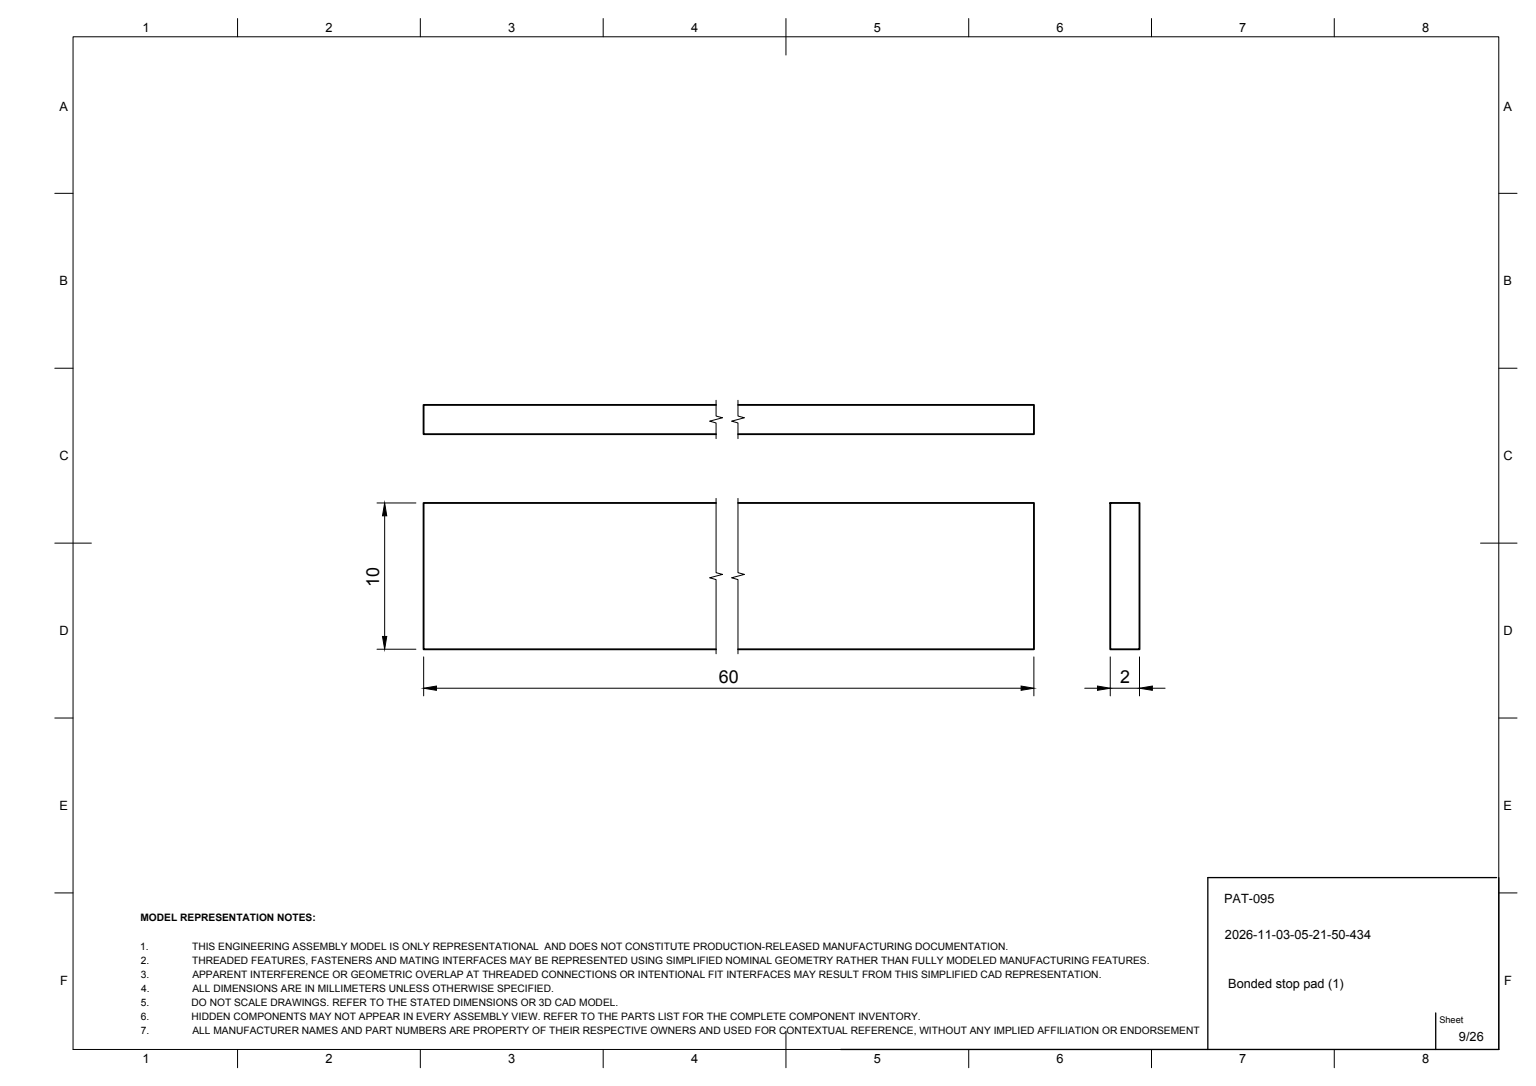
ISO-10303-21;
HEADER;
/* Generated by software containing ST-Developer
 * from STEP Tools, Inc. (www.steptools.com) 
 */

FILE_DESCRIPTION(
/* description */ ('Single-Axis Profile-Rail Linear Slide'),
/* implementation_level */ '2;1');

FILE_NAME(
/* name */ 'Bonded stop pad (1).step',
/* time_stamp */ '2026-10-27T10:47:43-07:00',
/* author */ (''),
/* organization */ (''),
/* preprocessor_version */ 'ST-DEVELOPER v20.2',
/* originating_system */ 'Autodesk Translation Framework v15.17.0.0',
/* authorisation */ '');

FILE_SCHEMA (('AUTOMOTIVE_DESIGN { 1 0 10303 214 3 1 1 }'));
ENDSEC;

DATA;
#10=MECHANICAL_DESIGN_GEOMETRIC_PRESENTATION_REPRESENTATION('',(#333),#14478);
#279=SHAPE_REPRESENTATION_RELATIONSHIP('SRR','None',#14609,#306);
#306=ADVANCED_BREP_SHAPE_REPRESENTATION('',(#360),#14453);
#333=STYLED_ITEM('',(#14845),#360);
#360=MANIFOLD_SOLID_BREP('Body1',#8593);
#496=PLANE('',#9020);
#497=PLANE('',#9021);
#498=PLANE('',#9022);
#499=PLANE('',#9023);
#500=PLANE('',#9024);
#501=PLANE('',#9025);
#890=FACE_OUTER_BOUND('',#1385,.T.);
#891=FACE_OUTER_BOUND('',#1386,.T.);
#892=FACE_OUTER_BOUND('',#1387,.T.);
#893=FACE_OUTER_BOUND('',#1388,.T.);
#894=FACE_OUTER_BOUND('',#1389,.T.);
#895=FACE_OUTER_BOUND('',#1390,.T.);
#1385=EDGE_LOOP('',(#6041,#6042,#6043,#6044));
#1386=EDGE_LOOP('',(#6045,#6046,#6047,#6048));
#1387=EDGE_LOOP('',(#6049,#6050,#6051,#6052));
#1388=EDGE_LOOP('',(#6053,#6054,#6055,#6056));
#1389=EDGE_LOOP('',(#6057,#6058,#6059,#6060));
#1390=EDGE_LOOP('',(#6061,#6062,#6063,#6064));
#1910=LINE('',#12246,#2881);
#1911=LINE('',#12248,#2882);
#1912=LINE('',#12250,#2883);
#1913=LINE('',#12251,#2884);
#1914=LINE('',#12254,#2885);
#1915=LINE('',#12256,#2886);
#1916=LINE('',#12257,#2887);
#1917=LINE('',#12260,#2888);
#1918=LINE('',#12262,#2889);
#1919=LINE('',#12263,#2890);
#1920=LINE('',#12265,#2891);
#1921=LINE('',#12266,#2892);
#2881=VECTOR('',#9895,1.);
#2882=VECTOR('',#9896,1.);
#2883=VECTOR('',#9897,1.);
#2884=VECTOR('',#9898,1.);
#2885=VECTOR('',#9901,1.);
#2886=VECTOR('',#9902,1.);
#2887=VECTOR('',#9903,1.);
#2888=VECTOR('',#9906,1.);
#2889=VECTOR('',#9907,1.);
#2890=VECTOR('',#9908,1.);
#2891=VECTOR('',#9911,1.);
#2892=VECTOR('',#9912,1.);
#4014=VERTEX_POINT('',#12244);
#4015=VERTEX_POINT('',#12245);
#4016=VERTEX_POINT('',#12247);
#4017=VERTEX_POINT('',#12249);
#4018=VERTEX_POINT('',#12253);
#4019=VERTEX_POINT('',#12255);
#4020=VERTEX_POINT('',#12259);
#4021=VERTEX_POINT('',#12261);
#4798=EDGE_CURVE('',#4014,#4015,#1910,.T.);
#4799=EDGE_CURVE('',#4015,#4016,#1911,.T.);
#4800=EDGE_CURVE('',#4017,#4016,#1912,.T.);
#4801=EDGE_CURVE('',#4014,#4017,#1913,.T.);
#4802=EDGE_CURVE('',#4018,#4014,#1914,.T.);
#4803=EDGE_CURVE('',#4019,#4017,#1915,.T.);
#4804=EDGE_CURVE('',#4018,#4019,#1916,.T.);
#4805=EDGE_CURVE('',#4020,#4018,#1917,.T.);
#4806=EDGE_CURVE('',#4021,#4019,#1918,.T.);
#4807=EDGE_CURVE('',#4020,#4021,#1919,.T.);
#4808=EDGE_CURVE('',#4015,#4020,#1920,.T.);
#4809=EDGE_CURVE('',#4016,#4021,#1921,.T.);
#6041=ORIENTED_EDGE('',*,*,#4798,.T.);
#6042=ORIENTED_EDGE('',*,*,#4799,.T.);
#6043=ORIENTED_EDGE('',*,*,#4800,.F.);
#6044=ORIENTED_EDGE('',*,*,#4801,.F.);
#6045=ORIENTED_EDGE('',*,*,#4802,.T.);
#6046=ORIENTED_EDGE('',*,*,#4801,.T.);
#6047=ORIENTED_EDGE('',*,*,#4803,.F.);
#6048=ORIENTED_EDGE('',*,*,#4804,.F.);
#6049=ORIENTED_EDGE('',*,*,#4805,.T.);
#6050=ORIENTED_EDGE('',*,*,#4804,.T.);
#6051=ORIENTED_EDGE('',*,*,#4806,.F.);
#6052=ORIENTED_EDGE('',*,*,#4807,.F.);
#6053=ORIENTED_EDGE('',*,*,#4808,.T.);
#6054=ORIENTED_EDGE('',*,*,#4807,.T.);
#6055=ORIENTED_EDGE('',*,*,#4809,.F.);
#6056=ORIENTED_EDGE('',*,*,#4799,.F.);
#6057=ORIENTED_EDGE('',*,*,#4809,.T.);
#6058=ORIENTED_EDGE('',*,*,#4806,.T.);
#6059=ORIENTED_EDGE('',*,*,#4803,.T.);
#6060=ORIENTED_EDGE('',*,*,#4800,.T.);
#6061=ORIENTED_EDGE('',*,*,#4808,.F.);
#6062=ORIENTED_EDGE('',*,*,#4798,.F.);
#6063=ORIENTED_EDGE('',*,*,#4802,.F.);
#6064=ORIENTED_EDGE('',*,*,#4805,.F.);
#8184=ADVANCED_FACE('',(#890),#496,.T.);
#8185=ADVANCED_FACE('',(#891),#497,.T.);
#8186=ADVANCED_FACE('',(#892),#498,.T.);
#8187=ADVANCED_FACE('',(#893),#499,.T.);
#8188=ADVANCED_FACE('',(#894),#500,.T.);
#8189=ADVANCED_FACE('',(#895),#501,.F.);
#8593=CLOSED_SHELL('',(#8184,#8185,#8186,#8187,#8188,#8189));
#9019=AXIS2_PLACEMENT_3D('',#12242,#9891,#9892);
#9020=AXIS2_PLACEMENT_3D('',#12243,#9893,#9894);
#9021=AXIS2_PLACEMENT_3D('',#12252,#9899,#9900);
#9022=AXIS2_PLACEMENT_3D('',#12258,#9904,#9905);
#9023=AXIS2_PLACEMENT_3D('',#12264,#9909,#9910);
#9024=AXIS2_PLACEMENT_3D('',#12267,#9913,#9914);
#9025=AXIS2_PLACEMENT_3D('',#12268,#9915,#9916);
#9891=DIRECTION('axis',(0.,0.,1.));
#9892=DIRECTION('refdir',(1.,0.,0.));
#9893=DIRECTION('center_axis',(0.,1.,0.));
#9894=DIRECTION('ref_axis',(-1.,0.,0.));
#9895=DIRECTION('',(-1.,0.,0.));
#9896=DIRECTION('',(0.,0.,1.));
#9897=DIRECTION('',(-1.,0.,0.));
#9898=DIRECTION('',(0.,0.,1.));
#9899=DIRECTION('center_axis',(1.,0.,0.));
#9900=DIRECTION('ref_axis',(0.,1.,0.));
#9901=DIRECTION('',(0.,1.,0.));
#9902=DIRECTION('',(0.,1.,0.));
#9903=DIRECTION('',(0.,0.,1.));
#9904=DIRECTION('center_axis',(0.,-1.,0.));
#9905=DIRECTION('ref_axis',(1.,0.,0.));
#9906=DIRECTION('',(1.,0.,0.));
#9907=DIRECTION('',(1.,0.,0.));
#9908=DIRECTION('',(0.,0.,1.));
#9909=DIRECTION('center_axis',(-1.,0.,0.));
#9910=DIRECTION('ref_axis',(0.,-1.,0.));
#9911=DIRECTION('',(0.,-1.,0.));
#9912=DIRECTION('',(0.,-1.,0.));
#9913=DIRECTION('center_axis',(0.,0.,1.));
#9914=DIRECTION('ref_axis',(1.,0.,0.));
#9915=DIRECTION('center_axis',(0.,0.,1.));
#9916=DIRECTION('ref_axis',(1.,0.,0.));
#12242=CARTESIAN_POINT('',(0.,0.,0.));
#12243=CARTESIAN_POINT('Origin',(22.,3.,5.2));
#12244=CARTESIAN_POINT('',(22.,3.,5.2));
#12245=CARTESIAN_POINT('',(21.8,3.,5.2));
#12246=CARTESIAN_POINT('',(22.,3.,5.2));
#12247=CARTESIAN_POINT('',(21.8,3.,6.2));
#12248=CARTESIAN_POINT('',(21.8,3.,5.2));
#12249=CARTESIAN_POINT('',(22.,3.,6.2));
#12250=CARTESIAN_POINT('',(22.,3.,6.2));
#12251=CARTESIAN_POINT('',(22.,3.,5.2));
#12252=CARTESIAN_POINT('Origin',(22.,-3.,5.2));
#12253=CARTESIAN_POINT('',(22.,-3.,5.2));
#12254=CARTESIAN_POINT('',(22.,-3.,5.2));
#12255=CARTESIAN_POINT('',(22.,-3.,6.2));
#12256=CARTESIAN_POINT('',(22.,-3.,6.2));
#12257=CARTESIAN_POINT('',(22.,-3.,5.2));
#12258=CARTESIAN_POINT('Origin',(21.8,-3.,5.2));
#12259=CARTESIAN_POINT('',(21.8,-3.,5.2));
#12260=CARTESIAN_POINT('',(21.8,-3.,5.2));
#12261=CARTESIAN_POINT('',(21.8,-3.,6.2));
#12262=CARTESIAN_POINT('',(21.8,-3.,6.2));
#12263=CARTESIAN_POINT('',(21.8,-3.,5.2));
#12264=CARTESIAN_POINT('Origin',(21.8,3.,5.2));
#12265=CARTESIAN_POINT('',(21.8,3.,5.2));
#12266=CARTESIAN_POINT('',(21.8,3.,6.2));
#12267=CARTESIAN_POINT('Origin',(21.9,0.,6.2));
#12268=CARTESIAN_POINT('Origin',(21.9,0.,5.2));
#14421=UNCERTAINTY_MEASURE_WITH_UNIT(LENGTH_MEASURE(0.001),#14479,
'DISTANCE_ACCURACY_VALUE',
'Maximum model space distance between geometric entities at asserted c
onnectivities');
#14446=UNCERTAINTY_MEASURE_WITH_UNIT(LENGTH_MEASURE(0.001),#14479,
'DISTANCE_ACCURACY_VALUE',
'Maximum model space distance between geometric entities at asserted c
onnectivities');
#14453=(
GEOMETRIC_REPRESENTATION_CONTEXT(3)
GLOBAL_UNCERTAINTY_ASSIGNED_CONTEXT((#14421))
GLOBAL_UNIT_ASSIGNED_CONTEXT((#14479,#14481,#14482))
REPRESENTATION_CONTEXT('','3D')
);
#14478=(
GEOMETRIC_REPRESENTATION_CONTEXT(3)
GLOBAL_UNCERTAINTY_ASSIGNED_CONTEXT((#14446))
GLOBAL_UNIT_ASSIGNED_CONTEXT((#14479,#14481,#14482))
REPRESENTATION_CONTEXT('','3D')
);
#14479=(
LENGTH_UNIT()
NAMED_UNIT(*)
SI_UNIT(.CENTI.,.METRE.)
);
#14481=(
NAMED_UNIT(*)
PLANE_ANGLE_UNIT()
SI_UNIT($,.RADIAN.)
);
#14482=(
NAMED_UNIT(*)
SI_UNIT($,.STERADIAN.)
SOLID_ANGLE_UNIT()
);
#14489=SHAPE_DEFINITION_REPRESENTATION(#14520,#14609);
#14520=PRODUCT_DEFINITION_SHAPE('',$,#14641);
#14609=SHAPE_REPRESENTATION('',(#9019),#14453);
#14634=PRODUCT_DEFINITION_CONTEXT('part definition',#14729,'design');
#14641=PRODUCT_DEFINITION('Bonded stop pad (1)','Bonded stop pad (1)',#14672,
#14634);
#14672=PRODUCT_DEFINITION_FORMATION('',$,#14737);
#14729=APPLICATION_CONTEXT(
'Core Data for Automotive Mechanical Design Process');
#14730=PRODUCT_CONTEXT('part definition',#14729,'mechanical');
#14737=PRODUCT('Bonded stop pad (1)','Bonded stop pad (1)',
'Bonded stop pad (1)',(#14730));
#14839=COLOUR_RGB('Off White',0.89,0.88,0.83);
#14840=FILL_AREA_STYLE_COLOUR('',#14839);
#14841=FILL_AREA_STYLE('',(#14840));
#14842=SURFACE_STYLE_FILL_AREA(#14841);
#14843=SURFACE_SIDE_STYLE('',(#14842));
#14844=SURFACE_STYLE_USAGE(.BOTH.,#14843);
#14845=PRESENTATION_STYLE_ASSIGNMENT((#14844));
ENDSEC;
END-ISO-10303-21;
